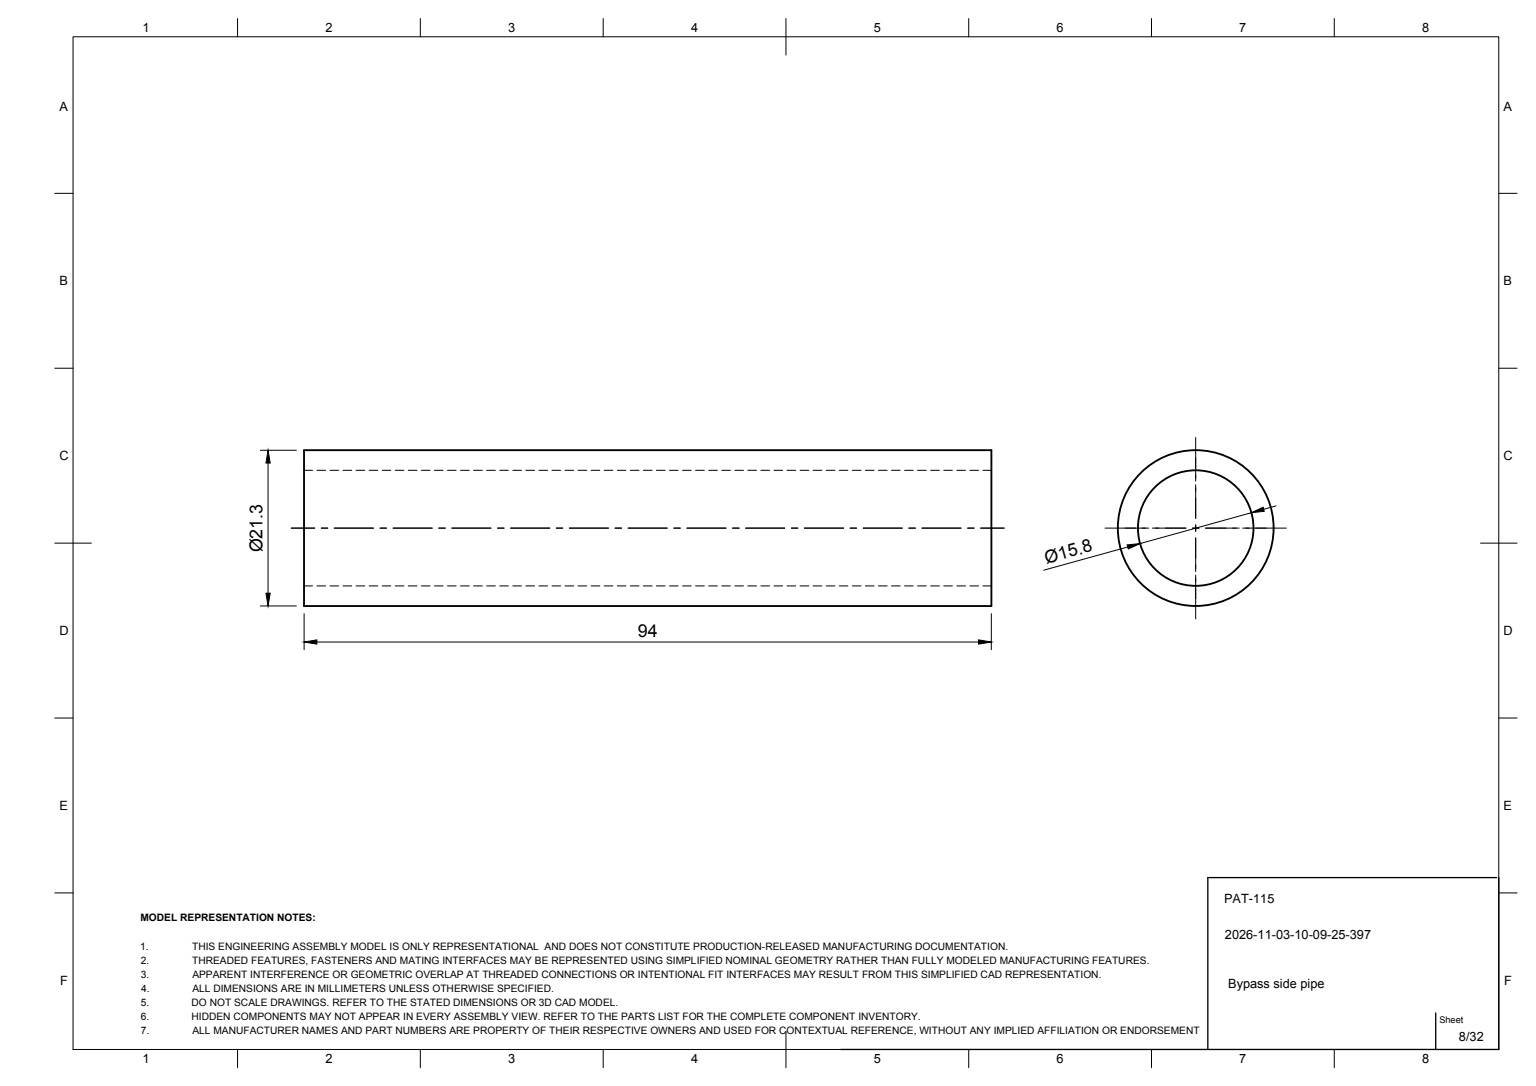
ISO-10303-21;
HEADER;
/* Generated by software containing ST-Developer
 * from STEP Tools, Inc. (www.steptools.com) 
 */

FILE_DESCRIPTION(
/* description */ ('Union bypass pipe loop'),
/* implementation_level */ '2;1');

FILE_NAME(
/* name */ 'Bypass side pipe.step',
/* time_stamp */ '2026-10-27T21:00:29-07:00',
/* author */ (''),
/* organization */ (''),
/* preprocessor_version */ 'ST-DEVELOPER v20.2',
/* originating_system */ 'Autodesk Translation Framework v15.17.0.0',
/* authorisation */ '');

FILE_SCHEMA (('AUTOMOTIVE_DESIGN { 1 0 10303 214 3 1 1 }'));
ENDSEC;

DATA;
#10=MECHANICAL_DESIGN_GEOMETRIC_PRESENTATION_REPRESENTATION('',(#462),#10095);
#398=SHAPE_REPRESENTATION_RELATIONSHIP('SRR','None',#10267,#430);
#430=ADVANCED_BREP_SHAPE_REPRESENTATION('',(#492),#10079);
#462=STYLED_ITEM('',(#10493),#492);
#492=MANIFOLD_SOLID_BREP('Body1',#5535);
#584=FACE_BOUND('',#1419,.T.);
#585=FACE_BOUND('',#1421,.T.);
#734=PLANE('',#6300);
#735=PLANE('',#6301);
#1011=FACE_OUTER_BOUND('',#1416,.T.);
#1012=FACE_OUTER_BOUND('',#1417,.T.);
#1013=FACE_OUTER_BOUND('',#1418,.T.);
#1014=FACE_OUTER_BOUND('',#1420,.T.);
#1416=EDGE_LOOP('',(#4452,#4453,#4454,#4455));
#1417=EDGE_LOOP('',(#4456,#4457,#4458,#4459));
#1418=EDGE_LOOP('',(#4460));
#1419=EDGE_LOOP('',(#4461));
#1420=EDGE_LOOP('',(#4462));
#1421=EDGE_LOOP('',(#4463));
#1811=LINE('',#9272,#2187);
#1812=LINE('',#9278,#2188);
#2187=VECTOR('',#7589,0.789999999999999);
#2188=VECTOR('',#7596,1.065);
#2518=CIRCLE('',#6295,0.789999999999999);
#2519=CIRCLE('',#6296,0.789999999999999);
#2520=CIRCLE('',#6298,1.065);
#2521=CIRCLE('',#6299,1.065);
#2862=VERTEX_POINT('',#9269);
#2863=VERTEX_POINT('',#9271);
#2864=VERTEX_POINT('',#9275);
#2865=VERTEX_POINT('',#9277);
#3424=EDGE_CURVE('',#2862,#2862,#2518,.T.);
#3425=EDGE_CURVE('',#2862,#2863,#1811,.T.);
#3426=EDGE_CURVE('',#2863,#2863,#2519,.T.);
#3427=EDGE_CURVE('',#2864,#2864,#2520,.T.);
#3428=EDGE_CURVE('',#2864,#2865,#1812,.T.);
#3429=EDGE_CURVE('',#2865,#2865,#2521,.T.);
#4452=ORIENTED_EDGE('',*,*,#3424,.F.);
#4453=ORIENTED_EDGE('',*,*,#3425,.T.);
#4454=ORIENTED_EDGE('',*,*,#3426,.T.);
#4455=ORIENTED_EDGE('',*,*,#3425,.F.);
#4456=ORIENTED_EDGE('',*,*,#3427,.F.);
#4457=ORIENTED_EDGE('',*,*,#3428,.T.);
#4458=ORIENTED_EDGE('',*,*,#3429,.T.);
#4459=ORIENTED_EDGE('',*,*,#3428,.F.);
#4460=ORIENTED_EDGE('',*,*,#3427,.T.);
#4461=ORIENTED_EDGE('',*,*,#3424,.T.);
#4462=ORIENTED_EDGE('',*,*,#3429,.F.);
#4463=ORIENTED_EDGE('',*,*,#3426,.F.);
#5143=CYLINDRICAL_SURFACE('',#6294,0.789999999999999);
#5144=CYLINDRICAL_SURFACE('',#6297,1.065);
#5360=ADVANCED_FACE('',(#1011),#5143,.F.);
#5361=ADVANCED_FACE('',(#1012),#5144,.T.);
#5362=ADVANCED_FACE('',(#1013,#584),#734,.T.);
#5363=ADVANCED_FACE('',(#1014,#585),#735,.F.);
#5535=CLOSED_SHELL('',(#5360,#5361,#5362,#5363));
#6293=AXIS2_PLACEMENT_3D('',#9267,#7583,#7584);
#6294=AXIS2_PLACEMENT_3D('',#9268,#7585,#7586);
#6295=AXIS2_PLACEMENT_3D('',#9270,#7587,#7588);
#6296=AXIS2_PLACEMENT_3D('',#9273,#7590,#7591);
#6297=AXIS2_PLACEMENT_3D('',#9274,#7592,#7593);
#6298=AXIS2_PLACEMENT_3D('',#9276,#7594,#7595);
#6299=AXIS2_PLACEMENT_3D('',#9279,#7597,#7598);
#6300=AXIS2_PLACEMENT_3D('',#9280,#7599,#7600);
#6301=AXIS2_PLACEMENT_3D('',#9281,#7601,#7602);
#7583=DIRECTION('axis',(0.,0.,1.));
#7584=DIRECTION('refdir',(1.,0.,0.));
#7585=DIRECTION('center_axis',(0.,1.,0.));
#7586=DIRECTION('ref_axis',(1.,0.,0.));
#7587=DIRECTION('center_axis',(0.,-1.,0.));
#7588=DIRECTION('ref_axis',(1.,0.,0.));
#7589=DIRECTION('',(0.,-1.,0.));
#7590=DIRECTION('center_axis',(0.,-1.,0.));
#7591=DIRECTION('ref_axis',(1.,0.,0.));
#7592=DIRECTION('center_axis',(0.,1.,0.));
#7593=DIRECTION('ref_axis',(1.,0.,0.));
#7594=DIRECTION('center_axis',(0.,1.,0.));
#7595=DIRECTION('ref_axis',(1.,0.,0.));
#7596=DIRECTION('',(0.,-1.,0.));
#7597=DIRECTION('center_axis',(0.,1.,0.));
#7598=DIRECTION('ref_axis',(1.,0.,0.));
#7599=DIRECTION('center_axis',(0.,1.,0.));
#7600=DIRECTION('ref_axis',(1.,0.,0.));
#7601=DIRECTION('center_axis',(0.,1.,0.));
#7602=DIRECTION('ref_axis',(1.,0.,0.));
#9267=CARTESIAN_POINT('',(0.,0.,0.));
#9268=CARTESIAN_POINT('Origin',(-12.,-10.5,5.));
#9269=CARTESIAN_POINT('',(-12.79,-1.1,5.));
#9270=CARTESIAN_POINT('Origin',(-12.,-1.1,5.));
#9271=CARTESIAN_POINT('',(-12.79,-10.5,5.));
#9272=CARTESIAN_POINT('',(-12.79,-10.5,5.));
#9273=CARTESIAN_POINT('Origin',(-12.,-10.5,5.));
#9274=CARTESIAN_POINT('Origin',(-12.,-10.5,5.));
#9275=CARTESIAN_POINT('',(-13.065,-1.1,5.));
#9276=CARTESIAN_POINT('Origin',(-12.,-1.1,5.));
#9277=CARTESIAN_POINT('',(-13.065,-10.5,5.));
#9278=CARTESIAN_POINT('',(-13.065,-10.5,5.));
#9279=CARTESIAN_POINT('Origin',(-12.,-10.5,5.));
#9280=CARTESIAN_POINT('Origin',(-12.,-1.1,5.));
#9281=CARTESIAN_POINT('Origin',(-12.,-10.5,5.));
#10042=UNCERTAINTY_MEASURE_WITH_UNIT(LENGTH_MEASURE(0.001),#10096,
'DISTANCE_ACCURACY_VALUE',
'Maximum model space distance between geometric entities at asserted c
onnectivities');
#10058=UNCERTAINTY_MEASURE_WITH_UNIT(LENGTH_MEASURE(0.001),#10096,
'DISTANCE_ACCURACY_VALUE',
'Maximum model space distance between geometric entities at asserted c
onnectivities');
#10079=(
GEOMETRIC_REPRESENTATION_CONTEXT(3)
GLOBAL_UNCERTAINTY_ASSIGNED_CONTEXT((#10042))
GLOBAL_UNIT_ASSIGNED_CONTEXT((#10096,#10098,#10099))
REPRESENTATION_CONTEXT('','3D')
);
#10095=(
GEOMETRIC_REPRESENTATION_CONTEXT(3)
GLOBAL_UNCERTAINTY_ASSIGNED_CONTEXT((#10058))
GLOBAL_UNIT_ASSIGNED_CONTEXT((#10096,#10098,#10099))
REPRESENTATION_CONTEXT('','3D')
);
#10096=(
LENGTH_UNIT()
NAMED_UNIT(*)
SI_UNIT(.CENTI.,.METRE.)
);
#10098=(
NAMED_UNIT(*)
PLANE_ANGLE_UNIT()
SI_UNIT($,.RADIAN.)
);
#10099=(
NAMED_UNIT(*)
SI_UNIT($,.STERADIAN.)
SOLID_ANGLE_UNIT()
);
#10120=SHAPE_DEFINITION_REPRESENTATION(#10191,#10267);
#10191=PRODUCT_DEFINITION_SHAPE('',$,#10304);
#10267=SHAPE_REPRESENTATION('',(#6293),#10079);
#10283=PRODUCT_DEFINITION_CONTEXT('part definition',#10393,'design');
#10304=PRODUCT_DEFINITION('Bypass side pipe','Bypass side pipe',#10340,
#10283);
#10340=PRODUCT_DEFINITION_FORMATION('',$,#10415);
#10393=APPLICATION_CONTEXT(
'Core Data for Automotive Mechanical Design Process');
#10394=PRODUCT_CONTEXT('part definition',#10393,'mechanical');
#10415=PRODUCT('Bypass side pipe','Bypass side pipe','Bypass side pipe',
(#10394));
#10487=COLOUR_RGB('Sky Blue',0.24,0.69,0.87);
#10488=FILL_AREA_STYLE_COLOUR('',#10487);
#10489=FILL_AREA_STYLE('',(#10488));
#10490=SURFACE_STYLE_FILL_AREA(#10489);
#10491=SURFACE_SIDE_STYLE('',(#10490));
#10492=SURFACE_STYLE_USAGE(.BOTH.,#10491);
#10493=PRESENTATION_STYLE_ASSIGNMENT((#10492));
ENDSEC;
END-ISO-10303-21;
